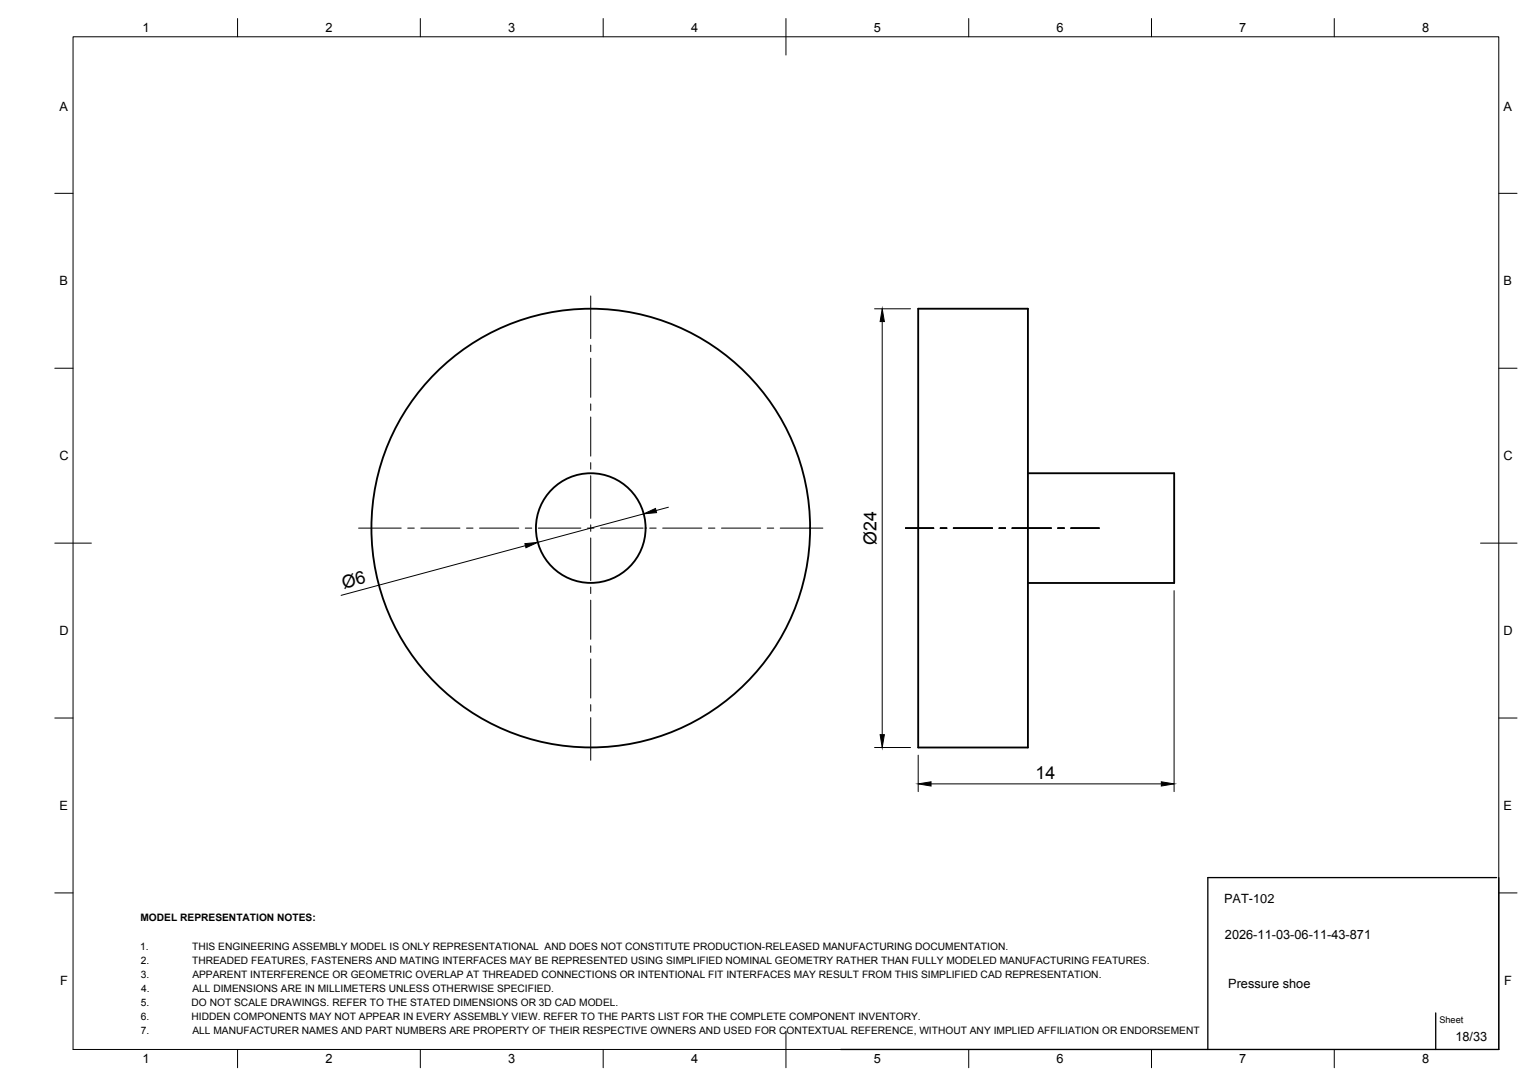
ISO-10303-21;
HEADER;
/* Generated by software containing ST-Developer
 * from STEP Tools, Inc. (www.steptools.com) 
 */

FILE_DESCRIPTION(
/* description */ ('Swing-away clamp arm'),
/* implementation_level */ '2;1');

FILE_NAME(
/* name */ 'Pressure shoe.step',
/* time_stamp */ '2026-10-28T03:26:03-07:00',
/* author */ (''),
/* organization */ (''),
/* preprocessor_version */ 'ST-DEVELOPER v20.2',
/* originating_system */ 'Autodesk Translation Framework v15.17.0.0',
/* authorisation */ '');

FILE_SCHEMA (('AUTOMOTIVE_DESIGN { 1 0 10303 214 3 1 1 }'));
ENDSEC;

DATA;
#10=MECHANICAL_DESIGN_GEOMETRIC_PRESENTATION_REPRESENTATION('',(#305),#10627);
#253=SHAPE_REPRESENTATION_RELATIONSHIP('SRR','None',#10752,#279);
#279=ADVANCED_BREP_SHAPE_REPRESENTATION('',(#338),#10611);
#305=STYLED_ITEM('',(#10951),#338);
#338=MANIFOLD_SOLID_BREP('Body1',#4912);
#431=FACE_BOUND('',#1199,.T.);
#573=PLANE('',#5567);
#574=PLANE('',#5571);
#575=PLANE('',#5572);
#815=FACE_OUTER_BOUND('',#1195,.T.);
#816=FACE_OUTER_BOUND('',#1196,.T.);
#817=FACE_OUTER_BOUND('',#1197,.T.);
#818=FACE_OUTER_BOUND('',#1198,.T.);
#819=FACE_OUTER_BOUND('',#1200,.T.);
#1195=EDGE_LOOP('',(#4023,#4024,#4025,#4026));
#1196=EDGE_LOOP('',(#4027));
#1197=EDGE_LOOP('',(#4028,#4029,#4030,#4031));
#1198=EDGE_LOOP('',(#4032));
#1199=EDGE_LOOP('',(#4033));
#1200=EDGE_LOOP('',(#4034));
#1583=LINE('',#9651,#1905);
#1584=LINE('',#9658,#1906);
#1905=VECTOR('',#6788,0.300000000000001);
#1906=VECTOR('',#6797,1.2);
#2133=CIRCLE('',#5565,0.300000000000001);
#2134=CIRCLE('',#5566,0.300000000000001);
#2135=CIRCLE('',#5569,1.2);
#2136=CIRCLE('',#5570,1.2);
#2508=VERTEX_POINT('',#9648);
#2509=VERTEX_POINT('',#9650);
#2510=VERTEX_POINT('',#9655);
#2511=VERTEX_POINT('',#9657);
#3044=EDGE_CURVE('',#2508,#2508,#2133,.T.);
#3045=EDGE_CURVE('',#2508,#2509,#1583,.T.);
#3046=EDGE_CURVE('',#2509,#2509,#2134,.T.);
#3047=EDGE_CURVE('',#2510,#2510,#2135,.T.);
#3048=EDGE_CURVE('',#2510,#2511,#1584,.T.);
#3049=EDGE_CURVE('',#2511,#2511,#2136,.T.);
#4023=ORIENTED_EDGE('',*,*,#3044,.F.);
#4024=ORIENTED_EDGE('',*,*,#3045,.T.);
#4025=ORIENTED_EDGE('',*,*,#3046,.F.);
#4026=ORIENTED_EDGE('',*,*,#3045,.F.);
#4027=ORIENTED_EDGE('',*,*,#3044,.T.);
#4028=ORIENTED_EDGE('',*,*,#3047,.F.);
#4029=ORIENTED_EDGE('',*,*,#3048,.T.);
#4030=ORIENTED_EDGE('',*,*,#3049,.T.);
#4031=ORIENTED_EDGE('',*,*,#3048,.F.);
#4032=ORIENTED_EDGE('',*,*,#3047,.T.);
#4033=ORIENTED_EDGE('',*,*,#3046,.T.);
#4034=ORIENTED_EDGE('',*,*,#3049,.F.);
#4556=CYLINDRICAL_SURFACE('',#5564,0.300000000000001);
#4557=CYLINDRICAL_SURFACE('',#5568,1.2);
#4770=ADVANCED_FACE('',(#815),#4556,.T.);
#4771=ADVANCED_FACE('',(#816),#573,.T.);
#4772=ADVANCED_FACE('',(#817),#4557,.T.);
#4773=ADVANCED_FACE('',(#818,#431),#574,.T.);
#4774=ADVANCED_FACE('',(#819),#575,.F.);
#4912=CLOSED_SHELL('',(#4770,#4771,#4772,#4773,#4774));
#5563=AXIS2_PLACEMENT_3D('',#9646,#6782,#6783);
#5564=AXIS2_PLACEMENT_3D('',#9647,#6784,#6785);
#5565=AXIS2_PLACEMENT_3D('',#9649,#6786,#6787);
#5566=AXIS2_PLACEMENT_3D('',#9652,#6789,#6790);
#5567=AXIS2_PLACEMENT_3D('',#9653,#6791,#6792);
#5568=AXIS2_PLACEMENT_3D('',#9654,#6793,#6794);
#5569=AXIS2_PLACEMENT_3D('',#9656,#6795,#6796);
#5570=AXIS2_PLACEMENT_3D('',#9659,#6798,#6799);
#5571=AXIS2_PLACEMENT_3D('',#9660,#6800,#6801);
#5572=AXIS2_PLACEMENT_3D('',#9661,#6802,#6803);
#6782=DIRECTION('axis',(0.,0.,1.));
#6783=DIRECTION('refdir',(1.,0.,0.));
#6784=DIRECTION('center_axis',(0.,0.,1.));
#6785=DIRECTION('ref_axis',(1.,0.,0.));
#6786=DIRECTION('center_axis',(0.,0.,1.));
#6787=DIRECTION('ref_axis',(1.,0.,0.));
#6788=DIRECTION('',(0.,0.,-1.));
#6789=DIRECTION('center_axis',(0.,0.,-1.));
#6790=DIRECTION('ref_axis',(1.,0.,0.));
#6791=DIRECTION('center_axis',(0.,0.,1.));
#6792=DIRECTION('ref_axis',(1.,0.,0.));
#6793=DIRECTION('center_axis',(0.,0.,1.));
#6794=DIRECTION('ref_axis',(1.,0.,0.));
#6795=DIRECTION('center_axis',(0.,0.,1.));
#6796=DIRECTION('ref_axis',(1.,0.,0.));
#6797=DIRECTION('',(0.,0.,-1.));
#6798=DIRECTION('center_axis',(0.,0.,1.));
#6799=DIRECTION('ref_axis',(1.,0.,0.));
#6800=DIRECTION('center_axis',(0.,0.,1.));
#6801=DIRECTION('ref_axis',(1.,0.,0.));
#6802=DIRECTION('center_axis',(0.,0.,1.));
#6803=DIRECTION('ref_axis',(1.,0.,0.));
#9646=CARTESIAN_POINT('',(0.,0.,0.));
#9647=CARTESIAN_POINT('Origin',(12.,0.,7.));
#9648=CARTESIAN_POINT('',(11.7,-3.67394039744207E-17,7.8));
#9649=CARTESIAN_POINT('Origin',(12.,0.,7.8));
#9650=CARTESIAN_POINT('',(11.7,-3.67394039744207E-17,7.));
#9651=CARTESIAN_POINT('',(11.7,-3.67394039744207E-17,7.));
#9652=CARTESIAN_POINT('Origin',(12.,0.,7.));
#9653=CARTESIAN_POINT('Origin',(12.,0.,7.8));
#9654=CARTESIAN_POINT('Origin',(12.,0.,6.4));
#9655=CARTESIAN_POINT('',(10.8,-1.46957615897682E-16,7.));
#9656=CARTESIAN_POINT('Origin',(12.,0.,7.));
#9657=CARTESIAN_POINT('',(10.8,-1.46957615897682E-16,6.4));
#9658=CARTESIAN_POINT('',(10.8,-1.46957615897682E-16,6.4));
#9659=CARTESIAN_POINT('Origin',(12.,0.,6.4));
#9660=CARTESIAN_POINT('Origin',(12.,0.,7.));
#9661=CARTESIAN_POINT('Origin',(12.,0.,6.4));
#10579=UNCERTAINTY_MEASURE_WITH_UNIT(LENGTH_MEASURE(0.001),#10628,
'DISTANCE_ACCURACY_VALUE',
'Maximum model space distance between geometric entities at asserted c
onnectivities');
#10595=UNCERTAINTY_MEASURE_WITH_UNIT(LENGTH_MEASURE(0.001),#10628,
'DISTANCE_ACCURACY_VALUE',
'Maximum model space distance between geometric entities at asserted c
onnectivities');
#10611=(
GEOMETRIC_REPRESENTATION_CONTEXT(3)
GLOBAL_UNCERTAINTY_ASSIGNED_CONTEXT((#10579))
GLOBAL_UNIT_ASSIGNED_CONTEXT((#10628,#10630,#10631))
REPRESENTATION_CONTEXT('','3D')
);
#10627=(
GEOMETRIC_REPRESENTATION_CONTEXT(3)
GLOBAL_UNCERTAINTY_ASSIGNED_CONTEXT((#10595))
GLOBAL_UNIT_ASSIGNED_CONTEXT((#10628,#10630,#10631))
REPRESENTATION_CONTEXT('','3D')
);
#10628=(
LENGTH_UNIT()
NAMED_UNIT(*)
SI_UNIT(.CENTI.,.METRE.)
);
#10630=(
NAMED_UNIT(*)
PLANE_ANGLE_UNIT()
SI_UNIT($,.RADIAN.)
);
#10631=(
NAMED_UNIT(*)
SI_UNIT($,.STERADIAN.)
SOLID_ANGLE_UNIT()
);
#10647=SHAPE_DEFINITION_REPRESENTATION(#10688,#10752);
#10688=PRODUCT_DEFINITION_SHAPE('',$,#10784);
#10752=SHAPE_REPRESENTATION('',(#5563),#10611);
#10768=PRODUCT_DEFINITION_CONTEXT('part definition',#10863,'design');
#10784=PRODUCT_DEFINITION('Pressure shoe','Pressure shoe',#10815,#10768);
#10815=PRODUCT_DEFINITION_FORMATION('',$,#10880);
#10863=APPLICATION_CONTEXT(
'Core Data for Automotive Mechanical Design Process');
#10864=PRODUCT_CONTEXT('part definition',#10863,'mechanical');
#10880=PRODUCT('Pressure shoe','Pressure shoe','Pressure shoe',(#10864));
#10945=COLOUR_RGB('Light Blue',0.38,0.62,0.78);
#10946=FILL_AREA_STYLE_COLOUR('',#10945);
#10947=FILL_AREA_STYLE('',(#10946));
#10948=SURFACE_STYLE_FILL_AREA(#10947);
#10949=SURFACE_SIDE_STYLE('',(#10948));
#10950=SURFACE_STYLE_USAGE(.BOTH.,#10949);
#10951=PRESENTATION_STYLE_ASSIGNMENT((#10950));
ENDSEC;
END-ISO-10303-21;
